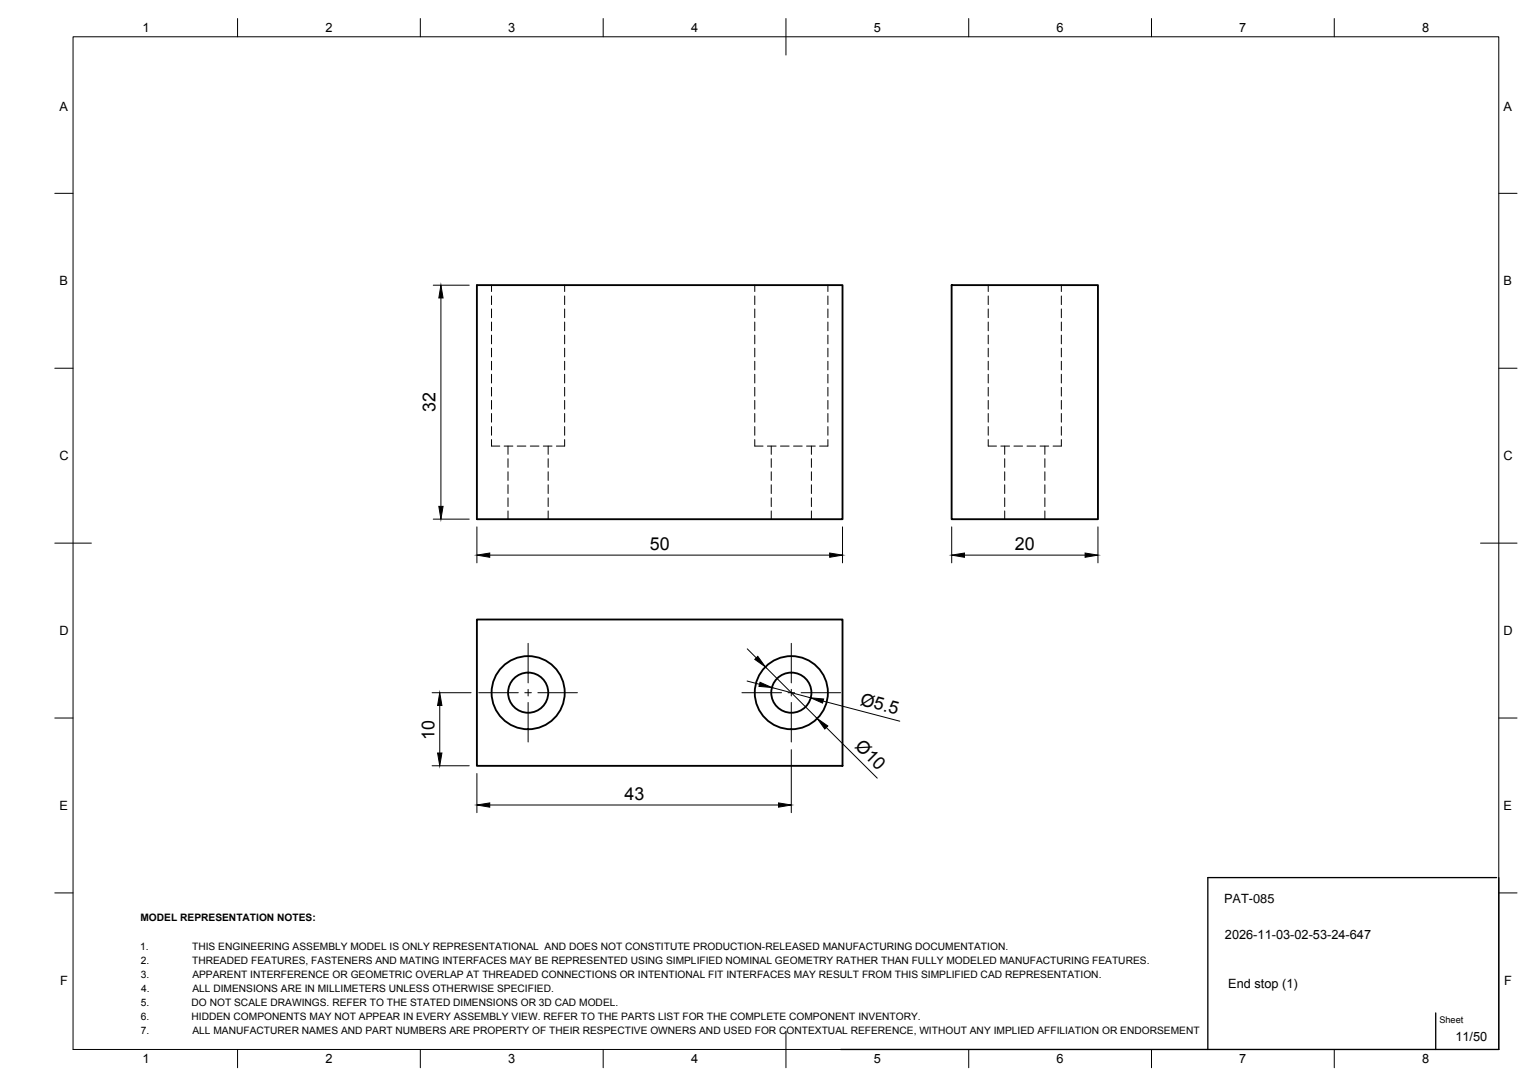
ISO-10303-21;
HEADER;
/* Generated by software containing ST-Developer
 * from STEP Tools, Inc. (www.steptools.com) 
 */

FILE_DESCRIPTION(
/* description */ ('Rack and pinion manual slide'),
/* implementation_level */ '2;1');

FILE_NAME(
/* name */ 'End stop (1).step',
/* time_stamp */ '2026-10-28T03:22:49-07:00',
/* author */ (''),
/* organization */ (''),
/* preprocessor_version */ 'ST-DEVELOPER v20.2',
/* originating_system */ 'Autodesk Translation Framework v15.17.0.0',
/* authorisation */ '');

FILE_SCHEMA (('AUTOMOTIVE_DESIGN { 1 0 10303 214 3 1 1 }'));
ENDSEC;

DATA;
#10=MECHANICAL_DESIGN_GEOMETRIC_PRESENTATION_REPRESENTATION('',(#738),#34851);
#646=SHAPE_REPRESENTATION_RELATIONSHIP('SRR','None',#35081,#692);
#692=ADVANCED_BREP_SHAPE_REPRESENTATION('',(#791),#34806);
#738=STYLED_ITEM('',(#35404),#791);
#791=MANIFOLD_SOLID_BREP('Body1',#13758);
#879=FACE_BOUND('',#2384,.T.);
#880=FACE_BOUND('',#2387,.T.);
#881=FACE_BOUND('',#2395,.T.);
#882=FACE_BOUND('',#2396,.T.);
#883=FACE_BOUND('',#2398,.T.);
#884=FACE_BOUND('',#2399,.T.);
#1082=PLANE('',#14439);
#1083=PLANE('',#14444);
#1084=PLANE('',#14450);
#1085=PLANE('',#14451);
#1086=PLANE('',#14452);
#1087=PLANE('',#14453);
#1088=PLANE('',#14454);
#1089=PLANE('',#14455);
#1597=FACE_OUTER_BOUND('',#2382,.T.);
#1598=FACE_OUTER_BOUND('',#2383,.T.);
#1599=FACE_OUTER_BOUND('',#2385,.T.);
#1600=FACE_OUTER_BOUND('',#2386,.T.);
#1601=FACE_OUTER_BOUND('',#2388,.T.);
#1602=FACE_OUTER_BOUND('',#2389,.T.);
#1603=FACE_OUTER_BOUND('',#2390,.T.);
#1604=FACE_OUTER_BOUND('',#2391,.T.);
#1605=FACE_OUTER_BOUND('',#2392,.T.);
#1606=FACE_OUTER_BOUND('',#2393,.T.);
#1607=FACE_OUTER_BOUND('',#2394,.T.);
#1608=FACE_OUTER_BOUND('',#2397,.T.);
#2382=EDGE_LOOP('',(#9522,#9523,#9524,#9525));
#2383=EDGE_LOOP('',(#9526));
#2384=EDGE_LOOP('',(#9527));
#2385=EDGE_LOOP('',(#9528,#9529,#9530,#9531));
#2386=EDGE_LOOP('',(#9532));
#2387=EDGE_LOOP('',(#9533));
#2388=EDGE_LOOP('',(#9534,#9535,#9536,#9537));
#2389=EDGE_LOOP('',(#9538,#9539,#9540,#9541));
#2390=EDGE_LOOP('',(#9542,#9543,#9544,#9545));
#2391=EDGE_LOOP('',(#9546,#9547,#9548,#9549));
#2392=EDGE_LOOP('',(#9550,#9551,#9552,#9553));
#2393=EDGE_LOOP('',(#9554,#9555,#9556,#9557));
#2394=EDGE_LOOP('',(#9558,#9559,#9560,#9561));
#2395=EDGE_LOOP('',(#9562));
#2396=EDGE_LOOP('',(#9563));
#2397=EDGE_LOOP('',(#9564,#9565,#9566,#9567));
#2398=EDGE_LOOP('',(#9568));
#2399=EDGE_LOOP('',(#9569));
#3320=LINE('',#19772,#4611);
#3321=LINE('',#19781,#4612);
#3322=LINE('',#19789,#4613);
#3323=LINE('',#19793,#4614);
#3324=LINE('',#19797,#4615);
#3325=LINE('',#19799,#4616);
#3326=LINE('',#19801,#4617);
#3327=LINE('',#19802,#4618);
#3328=LINE('',#19805,#4619);
#3329=LINE('',#19807,#4620);
#3330=LINE('',#19808,#4621);
#3331=LINE('',#19811,#4622);
#3332=LINE('',#19813,#4623);
#3333=LINE('',#19814,#4624);
#3334=LINE('',#19816,#4625);
#3335=LINE('',#19817,#4626);
#4611=VECTOR('',#15938,0.5);
#4612=VECTOR('',#15949,0.5);
#4613=VECTOR('',#15960,0.274999999999999);
#4614=VECTOR('',#15965,0.274999999999999);
#4615=VECTOR('',#15968,1.);
#4616=VECTOR('',#15969,1.);
#4617=VECTOR('',#15970,1.);
#4618=VECTOR('',#15971,1.);
#4619=VECTOR('',#15974,1.);
#4620=VECTOR('',#15975,1.);
#4621=VECTOR('',#15976,1.);
#4622=VECTOR('',#15979,1.);
#4623=VECTOR('',#15980,1.);
#4624=VECTOR('',#15981,1.);
#4625=VECTOR('',#15984,1.);
#4626=VECTOR('',#15985,1.);
#5854=CIRCLE('',#14437,0.5);
#5855=CIRCLE('',#14438,0.5);
#5856=CIRCLE('',#14440,0.274999999999999);
#5857=CIRCLE('',#14442,0.5);
#5858=CIRCLE('',#14443,0.5);
#5859=CIRCLE('',#14445,0.274999999999999);
#5860=CIRCLE('',#14447,0.274999999999999);
#5861=CIRCLE('',#14449,0.274999999999999);
#6320=VERTEX_POINT('',#19769);
#6321=VERTEX_POINT('',#19771);
#6322=VERTEX_POINT('',#19775);
#6323=VERTEX_POINT('',#19778);
#6324=VERTEX_POINT('',#19780);
#6325=VERTEX_POINT('',#19784);
#6326=VERTEX_POINT('',#19787);
#6327=VERTEX_POINT('',#19791);
#6328=VERTEX_POINT('',#19795);
#6329=VERTEX_POINT('',#19796);
#6330=VERTEX_POINT('',#19798);
#6331=VERTEX_POINT('',#19800);
#6332=VERTEX_POINT('',#19804);
#6333=VERTEX_POINT('',#19806);
#6334=VERTEX_POINT('',#19810);
#6335=VERTEX_POINT('',#19812);
#7573=EDGE_CURVE('',#6320,#6320,#5854,.T.);
#7574=EDGE_CURVE('',#6320,#6321,#3320,.T.);
#7575=EDGE_CURVE('',#6321,#6321,#5855,.T.);
#7576=EDGE_CURVE('',#6322,#6322,#5856,.T.);
#7577=EDGE_CURVE('',#6323,#6323,#5857,.T.);
#7578=EDGE_CURVE('',#6323,#6324,#3321,.T.);
#7579=EDGE_CURVE('',#6324,#6324,#5858,.T.);
#7580=EDGE_CURVE('',#6325,#6325,#5859,.T.);
#7581=EDGE_CURVE('',#6326,#6326,#5860,.T.);
#7582=EDGE_CURVE('',#6326,#6322,#3322,.T.);
#7583=EDGE_CURVE('',#6327,#6327,#5861,.T.);
#7584=EDGE_CURVE('',#6327,#6325,#3323,.T.);
#7585=EDGE_CURVE('',#6328,#6329,#3324,.T.);
#7586=EDGE_CURVE('',#6329,#6330,#3325,.T.);
#7587=EDGE_CURVE('',#6331,#6330,#3326,.T.);
#7588=EDGE_CURVE('',#6328,#6331,#3327,.T.);
#7589=EDGE_CURVE('',#6332,#6328,#3328,.T.);
#7590=EDGE_CURVE('',#6333,#6331,#3329,.T.);
#7591=EDGE_CURVE('',#6332,#6333,#3330,.T.);
#7592=EDGE_CURVE('',#6334,#6332,#3331,.T.);
#7593=EDGE_CURVE('',#6335,#6333,#3332,.T.);
#7594=EDGE_CURVE('',#6334,#6335,#3333,.T.);
#7595=EDGE_CURVE('',#6329,#6334,#3334,.T.);
#7596=EDGE_CURVE('',#6330,#6335,#3335,.T.);
#9522=ORIENTED_EDGE('',*,*,#7573,.F.);
#9523=ORIENTED_EDGE('',*,*,#7574,.T.);
#9524=ORIENTED_EDGE('',*,*,#7575,.F.);
#9525=ORIENTED_EDGE('',*,*,#7574,.F.);
#9526=ORIENTED_EDGE('',*,*,#7573,.T.);
#9527=ORIENTED_EDGE('',*,*,#7576,.F.);
#9528=ORIENTED_EDGE('',*,*,#7577,.F.);
#9529=ORIENTED_EDGE('',*,*,#7578,.T.);
#9530=ORIENTED_EDGE('',*,*,#7579,.F.);
#9531=ORIENTED_EDGE('',*,*,#7578,.F.);
#9532=ORIENTED_EDGE('',*,*,#7577,.T.);
#9533=ORIENTED_EDGE('',*,*,#7580,.F.);
#9534=ORIENTED_EDGE('',*,*,#7581,.F.);
#9535=ORIENTED_EDGE('',*,*,#7582,.T.);
#9536=ORIENTED_EDGE('',*,*,#7576,.T.);
#9537=ORIENTED_EDGE('',*,*,#7582,.F.);
#9538=ORIENTED_EDGE('',*,*,#7583,.F.);
#9539=ORIENTED_EDGE('',*,*,#7584,.T.);
#9540=ORIENTED_EDGE('',*,*,#7580,.T.);
#9541=ORIENTED_EDGE('',*,*,#7584,.F.);
#9542=ORIENTED_EDGE('',*,*,#7585,.T.);
#9543=ORIENTED_EDGE('',*,*,#7586,.T.);
#9544=ORIENTED_EDGE('',*,*,#7587,.F.);
#9545=ORIENTED_EDGE('',*,*,#7588,.F.);
#9546=ORIENTED_EDGE('',*,*,#7589,.T.);
#9547=ORIENTED_EDGE('',*,*,#7588,.T.);
#9548=ORIENTED_EDGE('',*,*,#7590,.F.);
#9549=ORIENTED_EDGE('',*,*,#7591,.F.);
#9550=ORIENTED_EDGE('',*,*,#7592,.T.);
#9551=ORIENTED_EDGE('',*,*,#7591,.T.);
#9552=ORIENTED_EDGE('',*,*,#7593,.F.);
#9553=ORIENTED_EDGE('',*,*,#7594,.F.);
#9554=ORIENTED_EDGE('',*,*,#7595,.T.);
#9555=ORIENTED_EDGE('',*,*,#7594,.T.);
#9556=ORIENTED_EDGE('',*,*,#7596,.F.);
#9557=ORIENTED_EDGE('',*,*,#7586,.F.);
#9558=ORIENTED_EDGE('',*,*,#7596,.T.);
#9559=ORIENTED_EDGE('',*,*,#7593,.T.);
#9560=ORIENTED_EDGE('',*,*,#7590,.T.);
#9561=ORIENTED_EDGE('',*,*,#7587,.T.);
#9562=ORIENTED_EDGE('',*,*,#7575,.T.);
#9563=ORIENTED_EDGE('',*,*,#7579,.T.);
#9564=ORIENTED_EDGE('',*,*,#7595,.F.);
#9565=ORIENTED_EDGE('',*,*,#7585,.F.);
#9566=ORIENTED_EDGE('',*,*,#7589,.F.);
#9567=ORIENTED_EDGE('',*,*,#7592,.F.);
#9568=ORIENTED_EDGE('',*,*,#7581,.T.);
#9569=ORIENTED_EDGE('',*,*,#7583,.T.);
#12868=CYLINDRICAL_SURFACE('',#14436,0.5);
#12869=CYLINDRICAL_SURFACE('',#14441,0.5);
#12870=CYLINDRICAL_SURFACE('',#14446,0.274999999999999);
#12871=CYLINDRICAL_SURFACE('',#14448,0.274999999999999);
#13075=ADVANCED_FACE('',(#1597),#12868,.F.);
#13076=ADVANCED_FACE('',(#1598,#879),#1082,.T.);
#13077=ADVANCED_FACE('',(#1599),#12869,.F.);
#13078=ADVANCED_FACE('',(#1600,#880),#1083,.T.);
#13079=ADVANCED_FACE('',(#1601),#12870,.F.);
#13080=ADVANCED_FACE('',(#1602),#12871,.F.);
#13081=ADVANCED_FACE('',(#1603),#1084,.T.);
#13082=ADVANCED_FACE('',(#1604),#1085,.T.);
#13083=ADVANCED_FACE('',(#1605),#1086,.T.);
#13084=ADVANCED_FACE('',(#1606),#1087,.T.);
#13085=ADVANCED_FACE('',(#1607,#881,#882),#1088,.T.);
#13086=ADVANCED_FACE('',(#1608,#883,#884),#1089,.F.);
#13758=CLOSED_SHELL('',(#13075,#13076,#13077,#13078,#13079,#13080,#13081,
#13082,#13083,#13084,#13085,#13086));
#14435=AXIS2_PLACEMENT_3D('',#19767,#15932,#15933);
#14436=AXIS2_PLACEMENT_3D('',#19768,#15934,#15935);
#14437=AXIS2_PLACEMENT_3D('',#19770,#15936,#15937);
#14438=AXIS2_PLACEMENT_3D('',#19773,#15939,#15940);
#14439=AXIS2_PLACEMENT_3D('',#19774,#15941,#15942);
#14440=AXIS2_PLACEMENT_3D('',#19776,#15943,#15944);
#14441=AXIS2_PLACEMENT_3D('',#19777,#15945,#15946);
#14442=AXIS2_PLACEMENT_3D('',#19779,#15947,#15948);
#14443=AXIS2_PLACEMENT_3D('',#19782,#15950,#15951);
#14444=AXIS2_PLACEMENT_3D('',#19783,#15952,#15953);
#14445=AXIS2_PLACEMENT_3D('',#19785,#15954,#15955);
#14446=AXIS2_PLACEMENT_3D('',#19786,#15956,#15957);
#14447=AXIS2_PLACEMENT_3D('',#19788,#15958,#15959);
#14448=AXIS2_PLACEMENT_3D('',#19790,#15961,#15962);
#14449=AXIS2_PLACEMENT_3D('',#19792,#15963,#15964);
#14450=AXIS2_PLACEMENT_3D('',#19794,#15966,#15967);
#14451=AXIS2_PLACEMENT_3D('',#19803,#15972,#15973);
#14452=AXIS2_PLACEMENT_3D('',#19809,#15977,#15978);
#14453=AXIS2_PLACEMENT_3D('',#19815,#15982,#15983);
#14454=AXIS2_PLACEMENT_3D('',#19818,#15986,#15987);
#14455=AXIS2_PLACEMENT_3D('',#19819,#15988,#15989);
#15932=DIRECTION('axis',(0.,0.,1.));
#15933=DIRECTION('refdir',(1.,0.,0.));
#15934=DIRECTION('center_axis',(0.,0.,1.));
#15935=DIRECTION('ref_axis',(1.,0.,0.));
#15936=DIRECTION('center_axis',(0.,0.,1.));
#15937=DIRECTION('ref_axis',(1.,0.,0.));
#15938=DIRECTION('',(0.,0.,1.));
#15939=DIRECTION('center_axis',(0.,0.,-1.));
#15940=DIRECTION('ref_axis',(1.,0.,0.));
#15941=DIRECTION('center_axis',(0.,0.,1.));
#15942=DIRECTION('ref_axis',(1.,0.,0.));
#15943=DIRECTION('center_axis',(0.,0.,1.));
#15944=DIRECTION('ref_axis',(1.,0.,0.));
#15945=DIRECTION('center_axis',(0.,0.,1.));
#15946=DIRECTION('ref_axis',(1.,0.,0.));
#15947=DIRECTION('center_axis',(0.,0.,1.));
#15948=DIRECTION('ref_axis',(1.,0.,0.));
#15949=DIRECTION('',(0.,0.,1.));
#15950=DIRECTION('center_axis',(0.,0.,-1.));
#15951=DIRECTION('ref_axis',(1.,0.,0.));
#15952=DIRECTION('center_axis',(0.,0.,1.));
#15953=DIRECTION('ref_axis',(1.,0.,0.));
#15954=DIRECTION('center_axis',(0.,0.,1.));
#15955=DIRECTION('ref_axis',(1.,0.,0.));
#15956=DIRECTION('center_axis',(0.,0.,1.));
#15957=DIRECTION('ref_axis',(1.,0.,0.));
#15958=DIRECTION('center_axis',(0.,0.,1.));
#15959=DIRECTION('ref_axis',(1.,0.,0.));
#15960=DIRECTION('',(0.,0.,1.));
#15961=DIRECTION('center_axis',(0.,0.,1.));
#15962=DIRECTION('ref_axis',(1.,0.,0.));
#15963=DIRECTION('center_axis',(0.,0.,1.));
#15964=DIRECTION('ref_axis',(1.,0.,0.));
#15965=DIRECTION('',(0.,0.,1.));
#15966=DIRECTION('center_axis',(0.,1.,0.));
#15967=DIRECTION('ref_axis',(-1.,0.,0.));
#15968=DIRECTION('',(-1.,0.,0.));
#15969=DIRECTION('',(0.,0.,1.));
#15970=DIRECTION('',(-1.,0.,0.));
#15971=DIRECTION('',(0.,0.,1.));
#15972=DIRECTION('center_axis',(1.,0.,0.));
#15973=DIRECTION('ref_axis',(0.,1.,0.));
#15974=DIRECTION('',(0.,1.,0.));
#15975=DIRECTION('',(0.,1.,0.));
#15976=DIRECTION('',(0.,0.,1.));
#15977=DIRECTION('center_axis',(0.,-1.,0.));
#15978=DIRECTION('ref_axis',(1.,0.,0.));
#15979=DIRECTION('',(1.,0.,0.));
#15980=DIRECTION('',(1.,0.,0.));
#15981=DIRECTION('',(0.,0.,1.));
#15982=DIRECTION('center_axis',(-1.,0.,0.));
#15983=DIRECTION('ref_axis',(0.,-1.,0.));
#15984=DIRECTION('',(0.,-1.,0.));
#15985=DIRECTION('',(0.,-1.,0.));
#15986=DIRECTION('center_axis',(0.,0.,1.));
#15987=DIRECTION('ref_axis',(1.,0.,0.));
#15988=DIRECTION('center_axis',(0.,0.,1.));
#15989=DIRECTION('ref_axis',(1.,0.,0.));
#19767=CARTESIAN_POINT('',(0.,0.,0.));
#19768=CARTESIAN_POINT('Origin',(26.2,-1.8,4.8));
#19769=CARTESIAN_POINT('',(25.7,-1.8,4.8));
#19770=CARTESIAN_POINT('Origin',(26.2,-1.8,4.8));
#19771=CARTESIAN_POINT('',(25.7,-1.8,7.));
#19772=CARTESIAN_POINT('',(25.7,-1.8,4.8));
#19773=CARTESIAN_POINT('Origin',(26.2,-1.8,7.));
#19774=CARTESIAN_POINT('Origin',(26.2,-1.8,4.8));
#19775=CARTESIAN_POINT('',(25.925,-1.8,4.8));
#19776=CARTESIAN_POINT('Origin',(26.2,-1.8,4.8));
#19777=CARTESIAN_POINT('Origin',(26.2,1.8,4.8));
#19778=CARTESIAN_POINT('',(25.7,1.8,4.8));
#19779=CARTESIAN_POINT('Origin',(26.2,1.8,4.8));
#19780=CARTESIAN_POINT('',(25.7,1.8,7.));
#19781=CARTESIAN_POINT('',(25.7,1.8,4.8));
#19782=CARTESIAN_POINT('Origin',(26.2,1.8,7.));
#19783=CARTESIAN_POINT('Origin',(26.2,1.8,4.8));
#19784=CARTESIAN_POINT('',(25.925,1.8,4.8));
#19785=CARTESIAN_POINT('Origin',(26.2,1.8,4.8));
#19786=CARTESIAN_POINT('Origin',(26.2,-1.8,3.7));
#19787=CARTESIAN_POINT('',(25.925,-1.8,3.8));
#19788=CARTESIAN_POINT('Origin',(26.2,-1.8,3.8));
#19789=CARTESIAN_POINT('',(25.925,-1.8,3.7));
#19790=CARTESIAN_POINT('Origin',(26.2,1.8,3.7));
#19791=CARTESIAN_POINT('',(25.925,1.8,3.8));
#19792=CARTESIAN_POINT('Origin',(26.2,1.8,3.8));
#19793=CARTESIAN_POINT('',(25.925,1.8,3.7));
#19794=CARTESIAN_POINT('Origin',(27.2,2.5,3.8));
#19795=CARTESIAN_POINT('',(27.2,2.5,3.8));
#19796=CARTESIAN_POINT('',(25.2,2.5,3.8));
#19797=CARTESIAN_POINT('',(27.2,2.5,3.8));
#19798=CARTESIAN_POINT('',(25.2,2.5,7.));
#19799=CARTESIAN_POINT('',(25.2,2.5,3.8));
#19800=CARTESIAN_POINT('',(27.2,2.5,7.));
#19801=CARTESIAN_POINT('',(27.2,2.5,7.));
#19802=CARTESIAN_POINT('',(27.2,2.5,3.8));
#19803=CARTESIAN_POINT('Origin',(27.2,-2.5,3.8));
#19804=CARTESIAN_POINT('',(27.2,-2.5,3.8));
#19805=CARTESIAN_POINT('',(27.2,-2.5,3.8));
#19806=CARTESIAN_POINT('',(27.2,-2.5,7.));
#19807=CARTESIAN_POINT('',(27.2,-2.5,7.));
#19808=CARTESIAN_POINT('',(27.2,-2.5,3.8));
#19809=CARTESIAN_POINT('Origin',(25.2,-2.5,3.8));
#19810=CARTESIAN_POINT('',(25.2,-2.5,3.8));
#19811=CARTESIAN_POINT('',(25.2,-2.5,3.8));
#19812=CARTESIAN_POINT('',(25.2,-2.5,7.));
#19813=CARTESIAN_POINT('',(25.2,-2.5,7.));
#19814=CARTESIAN_POINT('',(25.2,-2.5,3.8));
#19815=CARTESIAN_POINT('Origin',(25.2,2.5,3.8));
#19816=CARTESIAN_POINT('',(25.2,2.5,3.8));
#19817=CARTESIAN_POINT('',(25.2,2.5,7.));
#19818=CARTESIAN_POINT('Origin',(26.2,0.,7.));
#19819=CARTESIAN_POINT('Origin',(26.2,0.,3.8));
#34752=UNCERTAINTY_MEASURE_WITH_UNIT(LENGTH_MEASURE(0.001),#34852,
'DISTANCE_ACCURACY_VALUE',
'Maximum model space distance between geometric entities at asserted c
onnectivities');
#34797=UNCERTAINTY_MEASURE_WITH_UNIT(LENGTH_MEASURE(0.001),#34852,
'DISTANCE_ACCURACY_VALUE',
'Maximum model space distance between geometric entities at asserted c
onnectivities');
#34806=(
GEOMETRIC_REPRESENTATION_CONTEXT(3)
GLOBAL_UNCERTAINTY_ASSIGNED_CONTEXT((#34752))
GLOBAL_UNIT_ASSIGNED_CONTEXT((#34852,#34854,#34855))
REPRESENTATION_CONTEXT('','3D')
);
#34851=(
GEOMETRIC_REPRESENTATION_CONTEXT(3)
GLOBAL_UNCERTAINTY_ASSIGNED_CONTEXT((#34797))
GLOBAL_UNIT_ASSIGNED_CONTEXT((#34852,#34854,#34855))
REPRESENTATION_CONTEXT('','3D')
);
#34852=(
LENGTH_UNIT()
NAMED_UNIT(*)
SI_UNIT(.CENTI.,.METRE.)
);
#34854=(
NAMED_UNIT(*)
PLANE_ANGLE_UNIT()
SI_UNIT($,.RADIAN.)
);
#34855=(
NAMED_UNIT(*)
SI_UNIT($,.STERADIAN.)
SOLID_ANGLE_UNIT()
);
#34864=SHAPE_DEFINITION_REPRESENTATION(#34917,#35081);
#34917=PRODUCT_DEFINITION_SHAPE('',$,#35135);
#35081=SHAPE_REPRESENTATION('',(#14435),#34806);
#35126=PRODUCT_DEFINITION_CONTEXT('part definition',#35287,'design');
#35135=PRODUCT_DEFINITION('End stop (1)','End stop (1)',#35188,#35126);
#35188=PRODUCT_DEFINITION_FORMATION('',$,#35297);
#35287=APPLICATION_CONTEXT(
'Core Data for Automotive Mechanical Design Process');
#35288=PRODUCT_CONTEXT('part definition',#35287,'mechanical');
#35297=PRODUCT('End stop (1)','End stop (1)','End stop (1)',(#35288));
#35398=COLOUR_RGB('Sky Blue',0.24,0.69,0.87);
#35399=FILL_AREA_STYLE_COLOUR('',#35398);
#35400=FILL_AREA_STYLE('',(#35399));
#35401=SURFACE_STYLE_FILL_AREA(#35400);
#35402=SURFACE_SIDE_STYLE('',(#35401));
#35403=SURFACE_STYLE_USAGE(.BOTH.,#35402);
#35404=PRESENTATION_STYLE_ASSIGNMENT((#35403));
ENDSEC;
END-ISO-10303-21;
